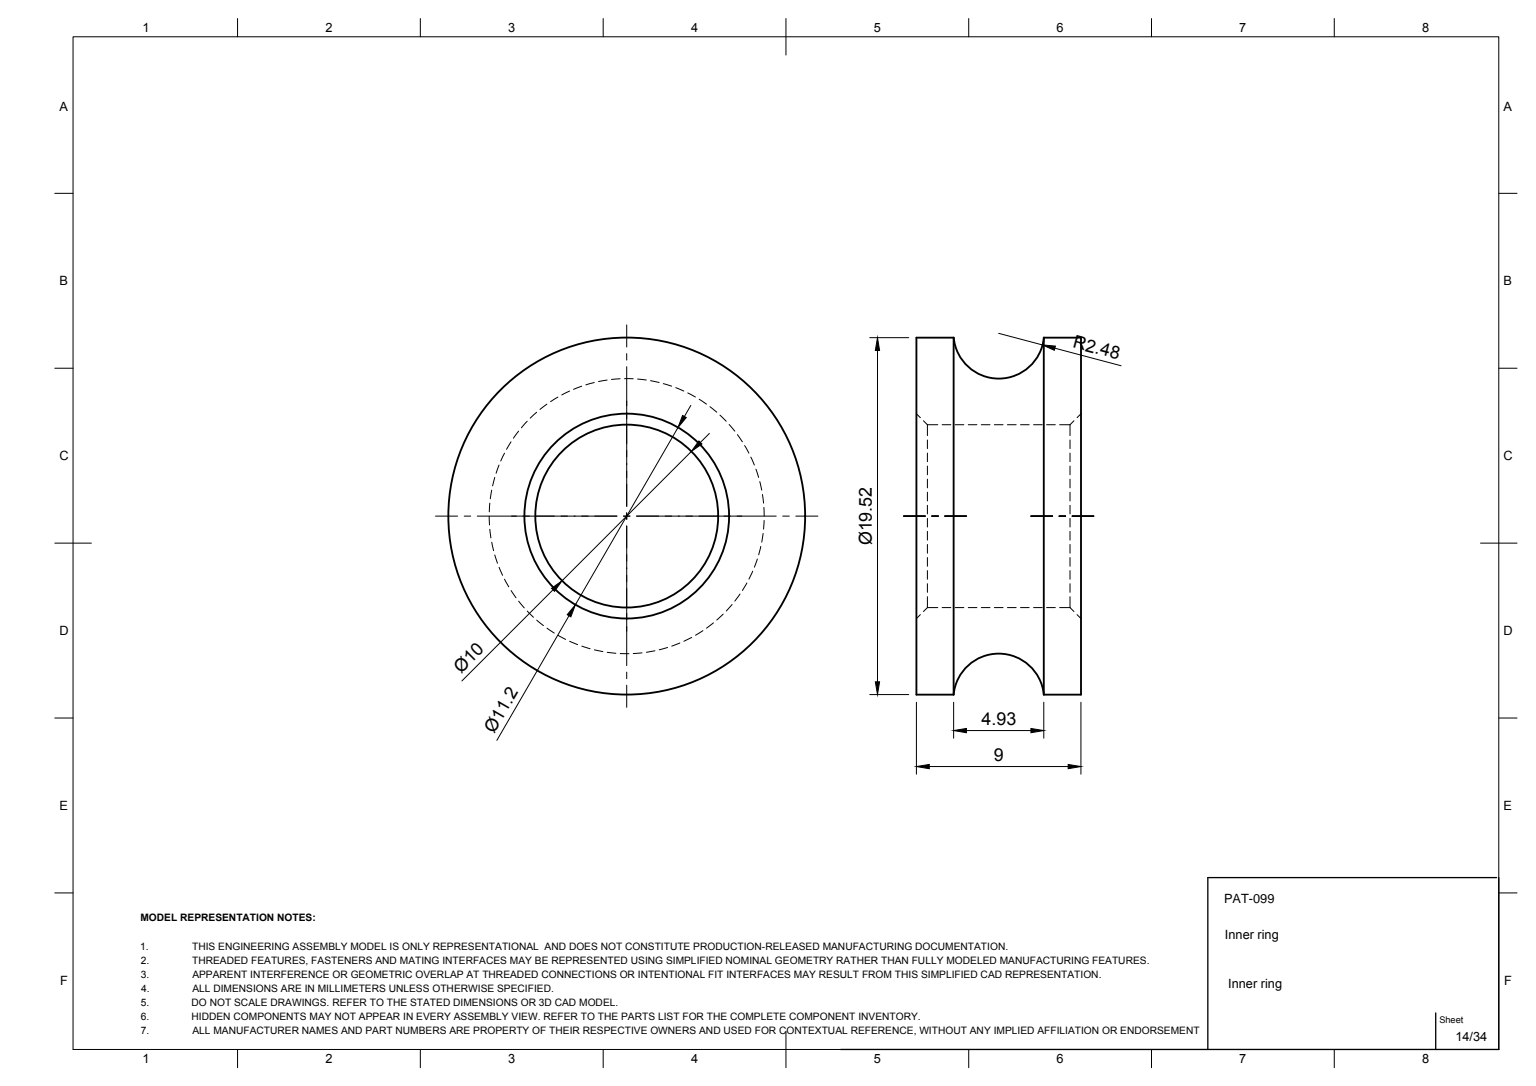
ISO-10303-21;
HEADER;
/* Generated by software containing ST-Developer
 * from STEP Tools, Inc. (www.steptools.com) 
 */

FILE_DESCRIPTION(
/* description */ ('PAT-099'),
/* implementation_level */ '2;1');

FILE_NAME(
/* name */ 'Inner ring.step',
/* time_stamp */ '2026-10-29T17:25:42-07:00',
/* author */ (''),
/* organization */ (''),
/* preprocessor_version */ 'ST-DEVELOPER v20.2',
/* originating_system */ 'Autodesk Translation Framework v15.17.0.0',
/* authorisation */ '');

FILE_SCHEMA (('AUTOMOTIVE_DESIGN { 1 0 10303 214 3 1 1 }'));
ENDSEC;

DATA;
#10=MECHANICAL_DESIGN_GEOMETRIC_PRESENTATION_REPRESENTATION('',(#357),#11035);
#27=TOROIDAL_SURFACE('',#5504,1.,0.247676);
#36=CONICAL_SURFACE('',#5515,0.53,0.785398163397448);
#37=CONICAL_SURFACE('',#5522,0.53,0.785398163397448);
#307=SHAPE_REPRESENTATION_RELATIONSHIP('SRR','None',#11180,#332);
#332=ADVANCED_BREP_SHAPE_REPRESENTATION('',(#388),#11030);
#357=STYLED_ITEM('',(#11386),#388);
#388=MANIFOLD_SOLID_BREP('Body1',#4727);
#514=FACE_BOUND('',#1288,.T.);
#515=FACE_BOUND('',#1291,.T.);
#642=PLANE('',#5517);
#643=PLANE('',#5520);
#889=FACE_OUTER_BOUND('',#1283,.T.);
#890=FACE_OUTER_BOUND('',#1284,.T.);
#891=FACE_OUTER_BOUND('',#1285,.T.);
#892=FACE_OUTER_BOUND('',#1286,.T.);
#893=FACE_OUTER_BOUND('',#1287,.T.);
#894=FACE_OUTER_BOUND('',#1289,.T.);
#895=FACE_OUTER_BOUND('',#1290,.T.);
#896=FACE_OUTER_BOUND('',#1292,.T.);
#1283=EDGE_LOOP('',(#4097,#4098,#4099,#4100,#4101,#4102));
#1284=EDGE_LOOP('',(#4103,#4104,#4105,#4106,#4107));
#1285=EDGE_LOOP('',(#4108,#4109,#4110,#4111));
#1286=EDGE_LOOP('',(#4112,#4113,#4114,#4115));
#1287=EDGE_LOOP('',(#4116));
#1288=EDGE_LOOP('',(#4117));
#1289=EDGE_LOOP('',(#4118,#4119,#4120,#4121,#4122));
#1290=EDGE_LOOP('',(#4123));
#1291=EDGE_LOOP('',(#4124));
#1292=EDGE_LOOP('',(#4125,#4126,#4127,#4128));
#1579=LINE('',#10366,#1831);
#1580=LINE('',#10372,#1832);
#1581=LINE('',#10376,#1833);
#1582=LINE('',#10382,#1834);
#1583=LINE('',#10387,#1835);
#1831=VECTOR('',#6894,0.976185);
#1832=VECTOR('',#6901,0.5);
#1833=VECTOR('',#6906,0.53);
#1834=VECTOR('',#6915,0.976185);
#1835=VECTOR('',#6922,0.53);
#2066=CIRCLE('',#5505,0.976185);
#2067=CIRCLE('',#5506,0.976185);
#2068=CIRCLE('',#5507,0.247676);
#2069=CIRCLE('',#5508,0.976185);
#2070=CIRCLE('',#5509,0.976185);
#2071=CIRCLE('',#5511,0.976185);
#2072=CIRCLE('',#5513,0.5);
#2073=CIRCLE('',#5514,0.5);
#2074=CIRCLE('',#5516,0.56);
#2075=CIRCLE('',#5519,0.976185);
#2076=CIRCLE('',#5521,0.56);
#2462=VERTEX_POINT('',#10355);
#2463=VERTEX_POINT('',#10356);
#2464=VERTEX_POINT('',#10359);
#2465=VERTEX_POINT('',#10361);
#2466=VERTEX_POINT('',#10365);
#2467=VERTEX_POINT('',#10369);
#2468=VERTEX_POINT('',#10371);
#2469=VERTEX_POINT('',#10375);
#2470=VERTEX_POINT('',#10380);
#2471=VERTEX_POINT('',#10384);
#3025=EDGE_CURVE('',#2462,#2463,#2066,.T.);
#3026=EDGE_CURVE('',#2463,#2462,#2067,.T.);
#3027=EDGE_CURVE('',#2463,#2464,#2068,.T.);
#3028=EDGE_CURVE('',#2465,#2464,#2069,.T.);
#3029=EDGE_CURVE('',#2464,#2465,#2070,.T.);
#3030=EDGE_CURVE('',#2465,#2466,#1579,.T.);
#3031=EDGE_CURVE('',#2466,#2466,#2071,.T.);
#3032=EDGE_CURVE('',#2467,#2467,#2072,.T.);
#3033=EDGE_CURVE('',#2467,#2468,#1580,.T.);
#3034=EDGE_CURVE('',#2468,#2468,#2073,.T.);
#3035=EDGE_CURVE('',#2468,#2469,#1581,.T.);
#3036=EDGE_CURVE('',#2469,#2469,#2074,.T.);
#3037=EDGE_CURVE('',#2470,#2470,#2075,.T.);
#3038=EDGE_CURVE('',#2470,#2462,#1582,.T.);
#3039=EDGE_CURVE('',#2471,#2471,#2076,.T.);
#3040=EDGE_CURVE('',#2471,#2467,#1583,.T.);
#4097=ORIENTED_EDGE('',*,*,#3025,.F.);
#4098=ORIENTED_EDGE('',*,*,#3026,.F.);
#4099=ORIENTED_EDGE('',*,*,#3027,.T.);
#4100=ORIENTED_EDGE('',*,*,#3028,.F.);
#4101=ORIENTED_EDGE('',*,*,#3029,.F.);
#4102=ORIENTED_EDGE('',*,*,#3027,.F.);
#4103=ORIENTED_EDGE('',*,*,#3028,.T.);
#4104=ORIENTED_EDGE('',*,*,#3029,.T.);
#4105=ORIENTED_EDGE('',*,*,#3030,.T.);
#4106=ORIENTED_EDGE('',*,*,#3031,.T.);
#4107=ORIENTED_EDGE('',*,*,#3030,.F.);
#4108=ORIENTED_EDGE('',*,*,#3032,.T.);
#4109=ORIENTED_EDGE('',*,*,#3033,.T.);
#4110=ORIENTED_EDGE('',*,*,#3034,.F.);
#4111=ORIENTED_EDGE('',*,*,#3033,.F.);
#4112=ORIENTED_EDGE('',*,*,#3034,.T.);
#4113=ORIENTED_EDGE('',*,*,#3035,.T.);
#4114=ORIENTED_EDGE('',*,*,#3036,.F.);
#4115=ORIENTED_EDGE('',*,*,#3035,.F.);
#4116=ORIENTED_EDGE('',*,*,#3031,.F.);
#4117=ORIENTED_EDGE('',*,*,#3036,.T.);
#4118=ORIENTED_EDGE('',*,*,#3037,.F.);
#4119=ORIENTED_EDGE('',*,*,#3038,.T.);
#4120=ORIENTED_EDGE('',*,*,#3025,.T.);
#4121=ORIENTED_EDGE('',*,*,#3026,.T.);
#4122=ORIENTED_EDGE('',*,*,#3038,.F.);
#4123=ORIENTED_EDGE('',*,*,#3037,.T.);
#4124=ORIENTED_EDGE('',*,*,#3039,.F.);
#4125=ORIENTED_EDGE('',*,*,#3039,.T.);
#4126=ORIENTED_EDGE('',*,*,#3040,.T.);
#4127=ORIENTED_EDGE('',*,*,#3032,.F.);
#4128=ORIENTED_EDGE('',*,*,#3040,.F.);
#4412=CYLINDRICAL_SURFACE('',#5510,0.976185);
#4413=CYLINDRICAL_SURFACE('',#5512,0.5);
#4414=CYLINDRICAL_SURFACE('',#5518,0.976185);
#4654=ADVANCED_FACE('',(#889),#27,.F.);
#4655=ADVANCED_FACE('',(#890),#4412,.T.);
#4656=ADVANCED_FACE('',(#891),#4413,.F.);
#4657=ADVANCED_FACE('',(#892),#36,.F.);
#4658=ADVANCED_FACE('',(#893,#514),#642,.T.);
#4659=ADVANCED_FACE('',(#894),#4414,.T.);
#4660=ADVANCED_FACE('',(#895,#515),#643,.T.);
#4661=ADVANCED_FACE('',(#896),#37,.F.);
#4727=CLOSED_SHELL('',(#4654,#4655,#4656,#4657,#4658,#4659,#4660,#4661));
#5503=AXIS2_PLACEMENT_3D('',#10353,#6878,#6879);
#5504=AXIS2_PLACEMENT_3D('',#10354,#6880,#6881);
#5505=AXIS2_PLACEMENT_3D('',#10357,#6882,#6883);
#5506=AXIS2_PLACEMENT_3D('',#10358,#6884,#6885);
#5507=AXIS2_PLACEMENT_3D('',#10360,#6886,#6887);
#5508=AXIS2_PLACEMENT_3D('',#10362,#6888,#6889);
#5509=AXIS2_PLACEMENT_3D('',#10363,#6890,#6891);
#5510=AXIS2_PLACEMENT_3D('',#10364,#6892,#6893);
#5511=AXIS2_PLACEMENT_3D('',#10367,#6895,#6896);
#5512=AXIS2_PLACEMENT_3D('',#10368,#6897,#6898);
#5513=AXIS2_PLACEMENT_3D('',#10370,#6899,#6900);
#5514=AXIS2_PLACEMENT_3D('',#10373,#6902,#6903);
#5515=AXIS2_PLACEMENT_3D('',#10374,#6904,#6905);
#5516=AXIS2_PLACEMENT_3D('',#10377,#6907,#6908);
#5517=AXIS2_PLACEMENT_3D('',#10378,#6909,#6910);
#5518=AXIS2_PLACEMENT_3D('',#10379,#6911,#6912);
#5519=AXIS2_PLACEMENT_3D('',#10381,#6913,#6914);
#5520=AXIS2_PLACEMENT_3D('',#10383,#6916,#6917);
#5521=AXIS2_PLACEMENT_3D('',#10385,#6918,#6919);
#5522=AXIS2_PLACEMENT_3D('',#10386,#6920,#6921);
#6878=DIRECTION('axis',(0.,0.,1.));
#6879=DIRECTION('refdir',(1.,0.,0.));
#6880=DIRECTION('center_axis',(0.,-1.,0.));
#6881=DIRECTION('ref_axis',(0.,0.,-1.));
#6882=DIRECTION('center_axis',(0.,-1.,0.));
#6883=DIRECTION('ref_axis',(1.,0.,0.));
#6884=DIRECTION('center_axis',(0.,-1.,0.));
#6885=DIRECTION('ref_axis',(1.,0.,0.));
#6886=DIRECTION('center_axis',(1.,0.,1.22464679914735E-16));
#6887=DIRECTION('ref_axis',(-1.22464679914735E-16,0.,1.));
#6888=DIRECTION('center_axis',(0.,1.,0.));
#6889=DIRECTION('ref_axis',(1.,0.,0.));
#6890=DIRECTION('center_axis',(0.,1.,0.));
#6891=DIRECTION('ref_axis',(1.,0.,0.));
#6892=DIRECTION('center_axis',(0.,-1.,0.));
#6893=DIRECTION('ref_axis',(1.,0.,0.));
#6894=DIRECTION('',(0.,1.,0.));
#6895=DIRECTION('center_axis',(0.,-1.,0.));
#6896=DIRECTION('ref_axis',(1.,0.,0.));
#6897=DIRECTION('center_axis',(0.,-1.,0.));
#6898=DIRECTION('ref_axis',(1.,0.,0.));
#6899=DIRECTION('center_axis',(0.,-1.,0.));
#6900=DIRECTION('ref_axis',(1.,0.,0.));
#6901=DIRECTION('',(0.,1.,0.));
#6902=DIRECTION('center_axis',(0.,-1.,0.));
#6903=DIRECTION('ref_axis',(1.,0.,0.));
#6904=DIRECTION('center_axis',(0.,1.,0.));
#6905=DIRECTION('ref_axis',(1.,0.,0.));
#6906=DIRECTION('',(-0.707106781186547,0.707106781186548,-8.65956056235493E-17));
#6907=DIRECTION('center_axis',(0.,-1.,0.));
#6908=DIRECTION('ref_axis',(1.,0.,0.));
#6909=DIRECTION('center_axis',(0.,1.,0.));
#6910=DIRECTION('ref_axis',(0.,0.,1.));
#6911=DIRECTION('center_axis',(0.,-1.,0.));
#6912=DIRECTION('ref_axis',(1.,0.,0.));
#6913=DIRECTION('center_axis',(0.,-1.,0.));
#6914=DIRECTION('ref_axis',(1.,0.,0.));
#6915=DIRECTION('',(0.,1.,0.));
#6916=DIRECTION('center_axis',(0.,-1.,0.));
#6917=DIRECTION('ref_axis',(0.,0.,-1.));
#6918=DIRECTION('center_axis',(0.,-1.,0.));
#6919=DIRECTION('ref_axis',(1.,0.,0.));
#6920=DIRECTION('center_axis',(0.,-1.,0.));
#6921=DIRECTION('ref_axis',(1.,0.,0.));
#6922=DIRECTION('',(0.707106781186547,0.707106781186548,8.65956056235493E-17));
#10353=CARTESIAN_POINT('',(0.,0.,0.));
#10354=CARTESIAN_POINT('Origin',(0.,0.,0.));
#10355=CARTESIAN_POINT('',(-0.976185,-0.246528389340863,-1.19548183562566E-16));
#10356=CARTESIAN_POINT('',(-1.19548183562566E-16,-0.246528389340863,0.976185));
#10357=CARTESIAN_POINT('Origin',(0.,-0.246528389340863,0.));
#10358=CARTESIAN_POINT('Origin',(0.,-0.246528389340863,0.));
#10359=CARTESIAN_POINT('',(-1.19548183562566E-16,0.246528389340863,0.976185));
#10360=CARTESIAN_POINT('Origin',(-1.22464679914735E-16,0.,1.));
#10361=CARTESIAN_POINT('',(-0.976185,0.246528389340863,1.19548183562566E-16));
#10362=CARTESIAN_POINT('Origin',(0.,0.246528389340863,0.));
#10363=CARTESIAN_POINT('Origin',(0.,0.246528389340863,0.));
#10364=CARTESIAN_POINT('Origin',(0.,0.,0.));
#10365=CARTESIAN_POINT('',(-0.976185,0.45,-1.19548183562566E-16));
#10366=CARTESIAN_POINT('',(-0.976185,0.,-1.19548183562566E-16));
#10367=CARTESIAN_POINT('Origin',(0.,0.45,0.));
#10368=CARTESIAN_POINT('Origin',(0.,0.,0.));
#10369=CARTESIAN_POINT('',(-0.5,-0.39,-6.12323399573677E-17));
#10370=CARTESIAN_POINT('Origin',(0.,-0.39,0.));
#10371=CARTESIAN_POINT('',(-0.5,0.39,-6.12323399573677E-17));
#10372=CARTESIAN_POINT('',(-0.5,0.,-6.12323399573677E-17));
#10373=CARTESIAN_POINT('Origin',(0.,0.39,0.));
#10374=CARTESIAN_POINT('Origin',(0.,0.42,0.));
#10375=CARTESIAN_POINT('',(-0.56,0.45,-6.85802207522518E-17));
#10376=CARTESIAN_POINT('',(-0.53,0.42,-6.49062803548097E-17));
#10377=CARTESIAN_POINT('Origin',(0.,0.45,0.));
#10378=CARTESIAN_POINT('Origin',(0.976185,0.45,0.));
#10379=CARTESIAN_POINT('Origin',(0.,0.,0.));
#10380=CARTESIAN_POINT('',(-0.976185,-0.45,-1.19548183562566E-16));
#10381=CARTESIAN_POINT('Origin',(0.,-0.45,0.));
#10382=CARTESIAN_POINT('',(-0.976185,0.,-1.19548183562566E-16));
#10383=CARTESIAN_POINT('Origin',(0.56,-0.45,0.));
#10384=CARTESIAN_POINT('',(-0.56,-0.45,-6.85802207522518E-17));
#10385=CARTESIAN_POINT('Origin',(0.,-0.45,0.));
#10386=CARTESIAN_POINT('Origin',(0.,-0.42,0.));
#10387=CARTESIAN_POINT('',(-0.53,-0.42,-6.49062803548097E-17));
#10997=UNCERTAINTY_MEASURE_WITH_UNIT(LENGTH_MEASURE(0.001),#11036,
'DISTANCE_ACCURACY_VALUE',
'Maximum model space distance between geometric entities at asserted c
onnectivities');
#11002=UNCERTAINTY_MEASURE_WITH_UNIT(LENGTH_MEASURE(0.001),#11036,
'DISTANCE_ACCURACY_VALUE',
'Maximum model space distance between geometric entities at asserted c
onnectivities');
#11030=(
GEOMETRIC_REPRESENTATION_CONTEXT(3)
GLOBAL_UNCERTAINTY_ASSIGNED_CONTEXT((#10997))
GLOBAL_UNIT_ASSIGNED_CONTEXT((#11036,#11038,#11039))
REPRESENTATION_CONTEXT('','3D')
);
#11035=(
GEOMETRIC_REPRESENTATION_CONTEXT(3)
GLOBAL_UNCERTAINTY_ASSIGNED_CONTEXT((#11002))
GLOBAL_UNIT_ASSIGNED_CONTEXT((#11036,#11038,#11039))
REPRESENTATION_CONTEXT('','3D')
);
#11036=(
LENGTH_UNIT()
NAMED_UNIT(*)
SI_UNIT(.CENTI.,.METRE.)
);
#11038=(
NAMED_UNIT(*)
PLANE_ANGLE_UNIT()
SI_UNIT($,.RADIAN.)
);
#11039=(
NAMED_UNIT(*)
SI_UNIT($,.STERADIAN.)
SOLID_ANGLE_UNIT()
);
#11067=SHAPE_DEFINITION_REPRESENTATION(#11111,#11180);
#11111=PRODUCT_DEFINITION_SHAPE('',$,#11213);
#11180=SHAPE_REPRESENTATION('',(#5503),#11030);
#11185=PRODUCT_DEFINITION_CONTEXT('part definition',#11283,'design');
#11213=PRODUCT_DEFINITION('Inner ring','Inner ring',#11245,#11185);
#11245=PRODUCT_DEFINITION_FORMATION('',$,#11312);
#11283=APPLICATION_CONTEXT(
'Core Data for Automotive Mechanical Design Process');
#11284=PRODUCT_CONTEXT('part definition',#11283,'mechanical');
#11312=PRODUCT('Inner ring','Inner ring','Inner ring',(#11284));
#11380=COLOUR_RGB('Grey',0.48,0.52,0.57);
#11381=FILL_AREA_STYLE_COLOUR('',#11380);
#11382=FILL_AREA_STYLE('',(#11381));
#11383=SURFACE_STYLE_FILL_AREA(#11382);
#11384=SURFACE_SIDE_STYLE('',(#11383));
#11385=SURFACE_STYLE_USAGE(.BOTH.,#11384);
#11386=PRESENTATION_STYLE_ASSIGNMENT((#11385));
ENDSEC;
END-ISO-10303-21;
